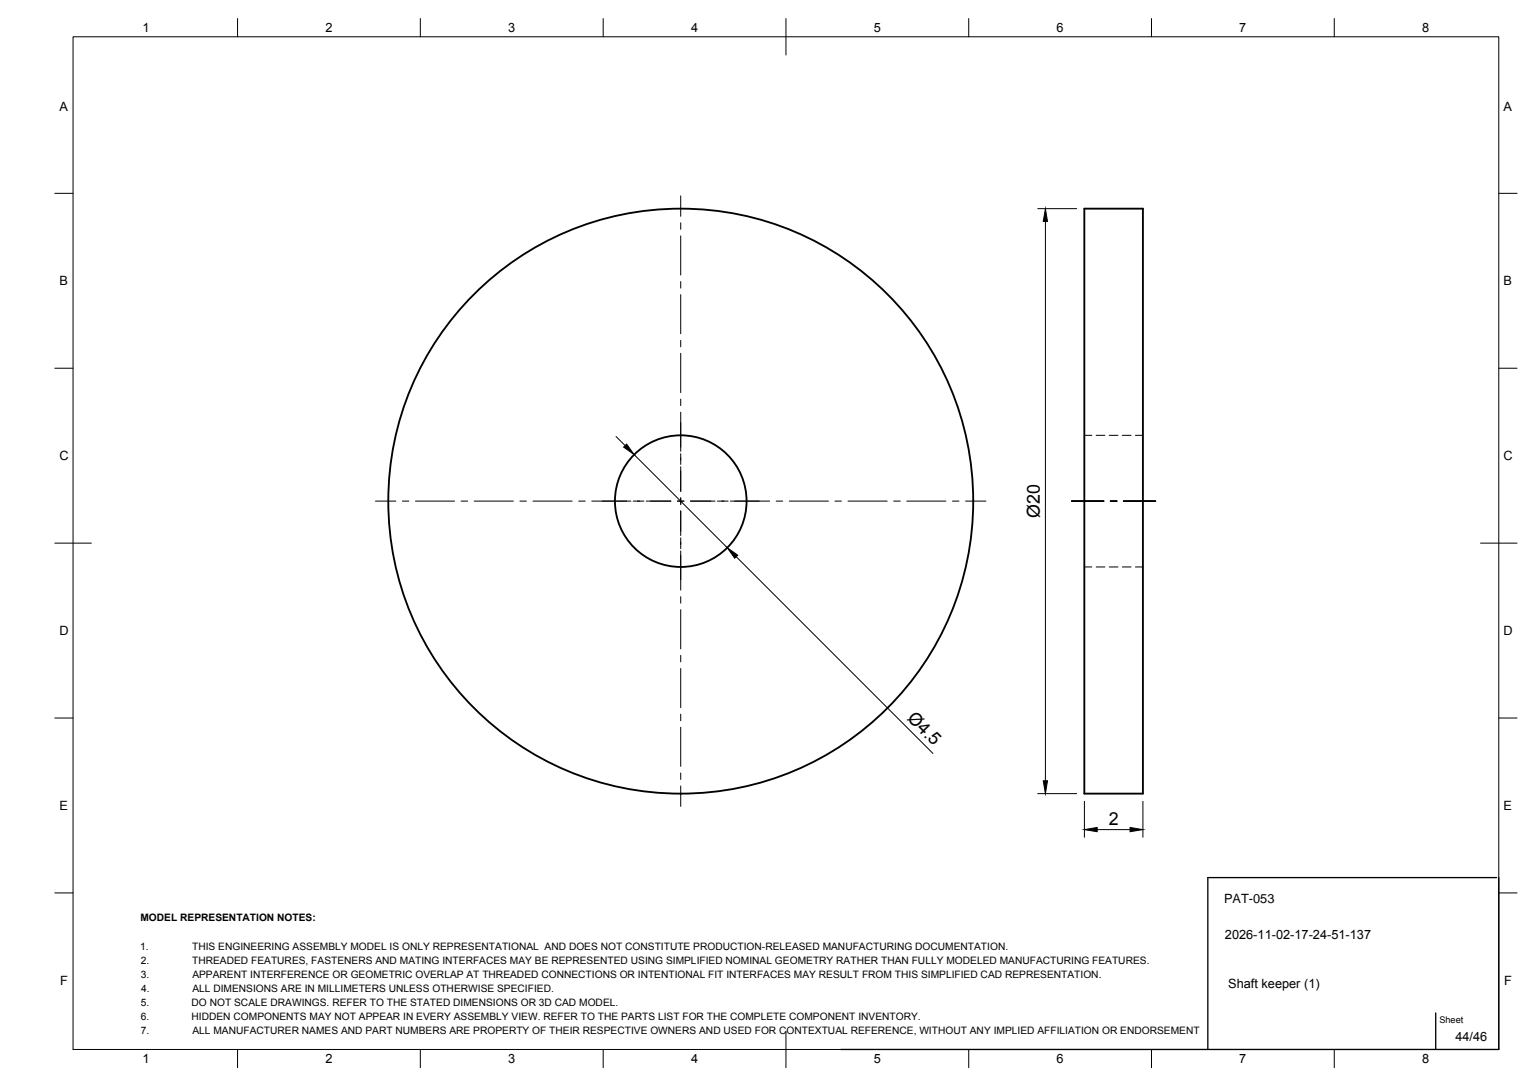
ISO-10303-21;
HEADER;
/* Generated by software containing ST-Developer
 * from STEP Tools, Inc. (www.steptools.com) 
 */

FILE_DESCRIPTION(
/* description */ ('Hand-operated arbor press'),
/* implementation_level */ '2;1');

FILE_NAME(
/* name */ 'Shaft keeper (1).step',
/* time_stamp */ '2026-10-28T03:25:25-07:00',
/* author */ (''),
/* organization */ (''),
/* preprocessor_version */ 'ST-DEVELOPER v20.2',
/* originating_system */ 'Autodesk Translation Framework v15.17.0.0',
/* authorisation */ '');

FILE_SCHEMA (('AUTOMOTIVE_DESIGN { 1 0 10303 214 3 1 1 }'));
ENDSEC;

DATA;
#10=MECHANICAL_DESIGN_GEOMETRIC_PRESENTATION_REPRESENTATION('',(#629),#32751);
#538=SHAPE_REPRESENTATION_RELATIONSHIP('SRR','None',#32970,#580);
#580=ADVANCED_BREP_SHAPE_REPRESENTATION('',(#676),#32744);
#629=STYLED_ITEM('',(#33242),#676);
#676=MANIFOLD_SOLID_BREP('Body1',#12528);
#838=FACE_BOUND('',#2682,.T.);
#839=FACE_BOUND('',#2684,.T.);
#1239=PLANE('',#13921);
#1240=PLANE('',#13922);
#1840=FACE_OUTER_BOUND('',#2679,.T.);
#1841=FACE_OUTER_BOUND('',#2680,.T.);
#1842=FACE_OUTER_BOUND('',#2681,.T.);
#1843=FACE_OUTER_BOUND('',#2683,.T.);
#2679=EDGE_LOOP('',(#10968,#10969,#10970,#10971));
#2680=EDGE_LOOP('',(#10972,#10973,#10974,#10975));
#2681=EDGE_LOOP('',(#10976));
#2682=EDGE_LOOP('',(#10977));
#2683=EDGE_LOOP('',(#10978));
#2684=EDGE_LOOP('',(#10979));
#3810=LINE('',#20811,#4981);
#3811=LINE('',#20817,#4982);
#4981=VECTOR('',#16977,0.225);
#4982=VECTOR('',#16984,1.);
#5484=CIRCLE('',#13916,0.225);
#5485=CIRCLE('',#13917,0.225);
#5486=CIRCLE('',#13919,1.);
#5487=CIRCLE('',#13920,1.);
#6443=VERTEX_POINT('',#20808);
#6444=VERTEX_POINT('',#20810);
#6445=VERTEX_POINT('',#20814);
#6446=VERTEX_POINT('',#20816);
#7987=EDGE_CURVE('',#6443,#6443,#5484,.T.);
#7988=EDGE_CURVE('',#6443,#6444,#3810,.T.);
#7989=EDGE_CURVE('',#6444,#6444,#5485,.T.);
#7990=EDGE_CURVE('',#6445,#6445,#5486,.T.);
#7991=EDGE_CURVE('',#6445,#6446,#3811,.T.);
#7992=EDGE_CURVE('',#6446,#6446,#5487,.T.);
#10968=ORIENTED_EDGE('',*,*,#7987,.F.);
#10969=ORIENTED_EDGE('',*,*,#7988,.T.);
#10970=ORIENTED_EDGE('',*,*,#7989,.T.);
#10971=ORIENTED_EDGE('',*,*,#7988,.F.);
#10972=ORIENTED_EDGE('',*,*,#7990,.F.);
#10973=ORIENTED_EDGE('',*,*,#7991,.T.);
#10974=ORIENTED_EDGE('',*,*,#7992,.T.);
#10975=ORIENTED_EDGE('',*,*,#7991,.F.);
#10976=ORIENTED_EDGE('',*,*,#7990,.T.);
#10977=ORIENTED_EDGE('',*,*,#7987,.T.);
#10978=ORIENTED_EDGE('',*,*,#7992,.F.);
#10979=ORIENTED_EDGE('',*,*,#7989,.F.);
#11770=CYLINDRICAL_SURFACE('',#13915,0.225);
#11771=CYLINDRICAL_SURFACE('',#13918,1.);
#12349=ADVANCED_FACE('',(#1840),#11770,.F.);
#12350=ADVANCED_FACE('',(#1841),#11771,.T.);
#12351=ADVANCED_FACE('',(#1842,#838),#1239,.T.);
#12352=ADVANCED_FACE('',(#1843,#839),#1240,.F.);
#12528=CLOSED_SHELL('',(#12349,#12350,#12351,#12352));
#13914=AXIS2_PLACEMENT_3D('',#20806,#16971,#16972);
#13915=AXIS2_PLACEMENT_3D('',#20807,#16973,#16974);
#13916=AXIS2_PLACEMENT_3D('',#20809,#16975,#16976);
#13917=AXIS2_PLACEMENT_3D('',#20812,#16978,#16979);
#13918=AXIS2_PLACEMENT_3D('',#20813,#16980,#16981);
#13919=AXIS2_PLACEMENT_3D('',#20815,#16982,#16983);
#13920=AXIS2_PLACEMENT_3D('',#20818,#16985,#16986);
#13921=AXIS2_PLACEMENT_3D('',#20819,#16987,#16988);
#13922=AXIS2_PLACEMENT_3D('',#20820,#16989,#16990);
#16971=DIRECTION('axis',(0.,0.,1.));
#16972=DIRECTION('refdir',(1.,0.,0.));
#16973=DIRECTION('center_axis',(0.,1.,0.));
#16974=DIRECTION('ref_axis',(1.,0.,0.));
#16975=DIRECTION('center_axis',(0.,-1.,0.));
#16976=DIRECTION('ref_axis',(1.,0.,0.));
#16977=DIRECTION('',(0.,-1.,0.));
#16978=DIRECTION('center_axis',(0.,-1.,0.));
#16979=DIRECTION('ref_axis',(1.,0.,0.));
#16980=DIRECTION('center_axis',(0.,1.,0.));
#16981=DIRECTION('ref_axis',(1.,0.,0.));
#16982=DIRECTION('center_axis',(0.,1.,0.));
#16983=DIRECTION('ref_axis',(1.,0.,0.));
#16984=DIRECTION('',(0.,-1.,0.));
#16985=DIRECTION('center_axis',(0.,1.,0.));
#16986=DIRECTION('ref_axis',(1.,0.,0.));
#16987=DIRECTION('center_axis',(0.,1.,0.));
#16988=DIRECTION('ref_axis',(1.,0.,0.));
#16989=DIRECTION('center_axis',(0.,1.,0.));
#16990=DIRECTION('ref_axis',(1.,0.,0.));
#20806=CARTESIAN_POINT('',(0.,0.,0.));
#20807=CARTESIAN_POINT('Origin',(-3.25,7.5,20.));
#20808=CARTESIAN_POINT('',(-3.475,7.7,20.));
#20809=CARTESIAN_POINT('Origin',(-3.25,7.7,20.));
#20810=CARTESIAN_POINT('',(-3.475,7.5,20.));
#20811=CARTESIAN_POINT('',(-3.475,7.5,20.));
#20812=CARTESIAN_POINT('Origin',(-3.25,7.5,20.));
#20813=CARTESIAN_POINT('Origin',(-3.25,7.5,20.));
#20814=CARTESIAN_POINT('',(-4.25,7.7,20.));
#20815=CARTESIAN_POINT('Origin',(-3.25,7.7,20.));
#20816=CARTESIAN_POINT('',(-4.25,7.5,20.));
#20817=CARTESIAN_POINT('',(-4.25,7.5,20.));
#20818=CARTESIAN_POINT('Origin',(-3.25,7.5,20.));
#20819=CARTESIAN_POINT('Origin',(-3.25,7.7,20.));
#20820=CARTESIAN_POINT('Origin',(-3.25,7.5,20.));
#32695=UNCERTAINTY_MEASURE_WITH_UNIT(LENGTH_MEASURE(0.001),#32752,
'DISTANCE_ACCURACY_VALUE',
'Maximum model space distance between geometric entities at asserted c
onnectivities');
#32702=UNCERTAINTY_MEASURE_WITH_UNIT(LENGTH_MEASURE(0.001),#32752,
'DISTANCE_ACCURACY_VALUE',
'Maximum model space distance between geometric entities at asserted c
onnectivities');
#32744=(
GEOMETRIC_REPRESENTATION_CONTEXT(3)
GLOBAL_UNCERTAINTY_ASSIGNED_CONTEXT((#32695))
GLOBAL_UNIT_ASSIGNED_CONTEXT((#32752,#32754,#32755))
REPRESENTATION_CONTEXT('','3D')
);
#32751=(
GEOMETRIC_REPRESENTATION_CONTEXT(3)
GLOBAL_UNCERTAINTY_ASSIGNED_CONTEXT((#32702))
GLOBAL_UNIT_ASSIGNED_CONTEXT((#32752,#32754,#32755))
REPRESENTATION_CONTEXT('','3D')
);
#32752=(
LENGTH_UNIT()
NAMED_UNIT(*)
SI_UNIT(.CENTI.,.METRE.)
);
#32754=(
NAMED_UNIT(*)
PLANE_ANGLE_UNIT()
SI_UNIT($,.RADIAN.)
);
#32755=(
NAMED_UNIT(*)
SI_UNIT($,.STERADIAN.)
SOLID_ANGLE_UNIT()
);
#32797=SHAPE_DEFINITION_REPRESENTATION(#32854,#32970);
#32854=PRODUCT_DEFINITION_SHAPE('',$,#33019);
#32970=SHAPE_REPRESENTATION('',(#13914),#32744);
#32977=PRODUCT_DEFINITION_CONTEXT('part definition',#33123,'design');
#33019=PRODUCT_DEFINITION('Shaft keeper (1)','Shaft keeper (1)',#33067,#32977);
#33067=PRODUCT_DEFINITION_FORMATION('',$,#33166);
#33123=APPLICATION_CONTEXT(
'Core Data for Automotive Mechanical Design Process');
#33124=PRODUCT_CONTEXT('part definition',#33123,'mechanical');
#33166=PRODUCT('Shaft keeper (1)','Shaft keeper (1)','Shaft keeper (1)',(#33124));
#33236=COLOUR_RGB('Grey',0.48,0.52,0.57);
#33237=FILL_AREA_STYLE_COLOUR('',#33236);
#33238=FILL_AREA_STYLE('',(#33237));
#33239=SURFACE_STYLE_FILL_AREA(#33238);
#33240=SURFACE_SIDE_STYLE('',(#33239));
#33241=SURFACE_STYLE_USAGE(.BOTH.,#33240);
#33242=PRESENTATION_STYLE_ASSIGNMENT((#33241));
ENDSEC;
END-ISO-10303-21;
